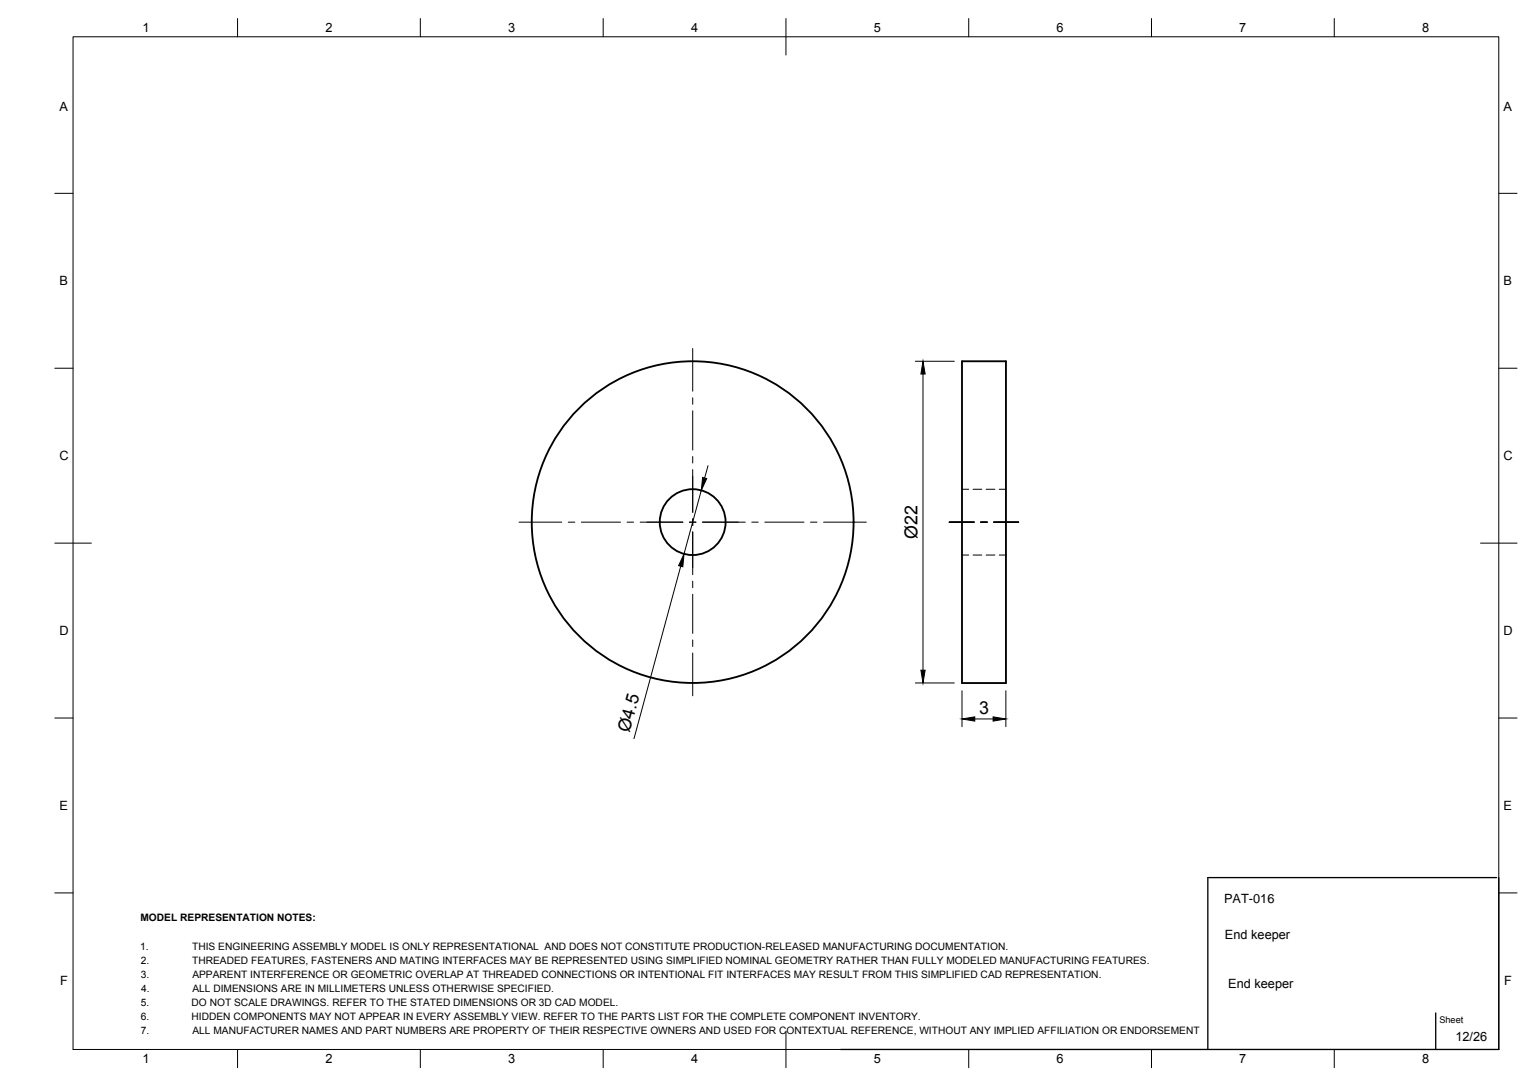
ISO-10303-21;
HEADER;
/* Generated by software containing ST-Developer
 * from STEP Tools, Inc. (www.steptools.com) 
 */

FILE_DESCRIPTION(
/* description */ ('Bracket-mounted idler roller'),
/* implementation_level */ '2;1');

FILE_NAME(
/* name */ 'End keeper.step',
/* time_stamp */ '2026-10-28T03:26:42-07:00',
/* author */ (''),
/* organization */ (''),
/* preprocessor_version */ 'ST-DEVELOPER v20.2',
/* originating_system */ 'Autodesk Translation Framework v15.17.0.0',
/* authorisation */ '');

FILE_SCHEMA (('AUTOMOTIVE_DESIGN { 1 0 10303 214 3 1 1 }'));
ENDSEC;

DATA;
#10=MECHANICAL_DESIGN_GEOMETRIC_PRESENTATION_REPRESENTATION('',(#289),#6241);
#247=SHAPE_REPRESENTATION_RELATIONSHIP('SRR','None',#6351,#268);
#268=ADVANCED_BREP_SHAPE_REPRESENTATION('',(#317),#6227);
#289=STYLED_ITEM('',(#6552),#317);
#317=MANIFOLD_SOLID_BREP('Body1',#3192);
#369=FACE_BOUND('',#826,.T.);
#370=FACE_BOUND('',#828,.T.);
#474=PLANE('',#3595);
#475=PLANE('',#3596);
#599=FACE_OUTER_BOUND('',#823,.T.);
#600=FACE_OUTER_BOUND('',#824,.T.);
#601=FACE_OUTER_BOUND('',#825,.T.);
#602=FACE_OUTER_BOUND('',#827,.T.);
#823=EDGE_LOOP('',(#2496,#2497,#2498,#2499));
#824=EDGE_LOOP('',(#2500,#2501,#2502,#2503));
#825=EDGE_LOOP('',(#2504));
#826=EDGE_LOOP('',(#2505));
#827=EDGE_LOOP('',(#2506));
#828=EDGE_LOOP('',(#2507));
#1095=LINE('',#5323,#1277);
#1096=LINE('',#5329,#1278);
#1277=VECTOR('',#4294,0.225);
#1278=VECTOR('',#4301,1.1);
#1392=CIRCLE('',#3590,0.225);
#1393=CIRCLE('',#3591,0.225);
#1394=CIRCLE('',#3593,1.1);
#1395=CIRCLE('',#3594,1.1);
#1633=VERTEX_POINT('',#5320);
#1634=VERTEX_POINT('',#5322);
#1635=VERTEX_POINT('',#5326);
#1636=VERTEX_POINT('',#5328);
#1950=EDGE_CURVE('',#1633,#1633,#1392,.T.);
#1951=EDGE_CURVE('',#1633,#1634,#1095,.T.);
#1952=EDGE_CURVE('',#1634,#1634,#1393,.T.);
#1953=EDGE_CURVE('',#1635,#1635,#1394,.T.);
#1954=EDGE_CURVE('',#1635,#1636,#1096,.T.);
#1955=EDGE_CURVE('',#1636,#1636,#1395,.T.);
#2496=ORIENTED_EDGE('',*,*,#1950,.F.);
#2497=ORIENTED_EDGE('',*,*,#1951,.T.);
#2498=ORIENTED_EDGE('',*,*,#1952,.T.);
#2499=ORIENTED_EDGE('',*,*,#1951,.F.);
#2500=ORIENTED_EDGE('',*,*,#1953,.F.);
#2501=ORIENTED_EDGE('',*,*,#1954,.T.);
#2502=ORIENTED_EDGE('',*,*,#1955,.T.);
#2503=ORIENTED_EDGE('',*,*,#1954,.F.);
#2504=ORIENTED_EDGE('',*,*,#1953,.T.);
#2505=ORIENTED_EDGE('',*,*,#1950,.T.);
#2506=ORIENTED_EDGE('',*,*,#1955,.F.);
#2507=ORIENTED_EDGE('',*,*,#1952,.F.);
#2951=CYLINDRICAL_SURFACE('',#3589,0.225);
#2952=CYLINDRICAL_SURFACE('',#3592,1.1);
#3074=ADVANCED_FACE('',(#599),#2951,.F.);
#3075=ADVANCED_FACE('',(#600),#2952,.T.);
#3076=ADVANCED_FACE('',(#601,#369),#474,.T.);
#3077=ADVANCED_FACE('',(#602,#370),#475,.F.);
#3192=CLOSED_SHELL('',(#3074,#3075,#3076,#3077));
#3588=AXIS2_PLACEMENT_3D('',#5318,#4288,#4289);
#3589=AXIS2_PLACEMENT_3D('',#5319,#4290,#4291);
#3590=AXIS2_PLACEMENT_3D('',#5321,#4292,#4293);
#3591=AXIS2_PLACEMENT_3D('',#5324,#4295,#4296);
#3592=AXIS2_PLACEMENT_3D('',#5325,#4297,#4298);
#3593=AXIS2_PLACEMENT_3D('',#5327,#4299,#4300);
#3594=AXIS2_PLACEMENT_3D('',#5330,#4302,#4303);
#3595=AXIS2_PLACEMENT_3D('',#5331,#4304,#4305);
#3596=AXIS2_PLACEMENT_3D('',#5332,#4306,#4307);
#4288=DIRECTION('axis',(0.,0.,1.));
#4289=DIRECTION('refdir',(1.,0.,0.));
#4290=DIRECTION('center_axis',(0.,1.,0.));
#4291=DIRECTION('ref_axis',(1.,0.,0.));
#4292=DIRECTION('center_axis',(0.,-1.,0.));
#4293=DIRECTION('ref_axis',(1.,0.,0.));
#4294=DIRECTION('',(0.,-1.,0.));
#4295=DIRECTION('center_axis',(0.,-1.,0.));
#4296=DIRECTION('ref_axis',(1.,0.,0.));
#4297=DIRECTION('center_axis',(0.,1.,0.));
#4298=DIRECTION('ref_axis',(1.,0.,0.));
#4299=DIRECTION('center_axis',(0.,1.,0.));
#4300=DIRECTION('ref_axis',(1.,0.,0.));
#4301=DIRECTION('',(0.,-1.,0.));
#4302=DIRECTION('center_axis',(0.,1.,0.));
#4303=DIRECTION('ref_axis',(1.,0.,0.));
#4304=DIRECTION('center_axis',(0.,1.,0.));
#4305=DIRECTION('ref_axis',(1.,0.,0.));
#4306=DIRECTION('center_axis',(0.,1.,0.));
#4307=DIRECTION('ref_axis',(1.,0.,0.));
#5318=CARTESIAN_POINT('',(0.,0.,0.));
#5319=CARTESIAN_POINT('Origin',(0.,-2.8,4.5));
#5320=CARTESIAN_POINT('',(-0.225,-2.5,4.5));
#5321=CARTESIAN_POINT('Origin',(0.,-2.5,4.5));
#5322=CARTESIAN_POINT('',(-0.225,-2.8,4.5));
#5323=CARTESIAN_POINT('',(-0.225,-2.8,4.5));
#5324=CARTESIAN_POINT('Origin',(0.,-2.8,4.5));
#5325=CARTESIAN_POINT('Origin',(0.,-2.8,4.5));
#5326=CARTESIAN_POINT('',(-1.1,-2.5,4.5));
#5327=CARTESIAN_POINT('Origin',(0.,-2.5,4.5));
#5328=CARTESIAN_POINT('',(-1.1,-2.8,4.5));
#5329=CARTESIAN_POINT('',(-1.1,-2.8,4.5));
#5330=CARTESIAN_POINT('Origin',(0.,-2.8,4.5));
#5331=CARTESIAN_POINT('Origin',(0.,-2.5,4.5));
#5332=CARTESIAN_POINT('Origin',(0.,-2.8,4.5));
#6201=UNCERTAINTY_MEASURE_WITH_UNIT(LENGTH_MEASURE(0.001),#6242,
'DISTANCE_ACCURACY_VALUE',
'Maximum model space distance between geometric entities at asserted c
onnectivities');
#6215=UNCERTAINTY_MEASURE_WITH_UNIT(LENGTH_MEASURE(0.001),#6242,
'DISTANCE_ACCURACY_VALUE',
'Maximum model space distance between geometric entities at asserted c
onnectivities');
#6227=(
GEOMETRIC_REPRESENTATION_CONTEXT(3)
GLOBAL_UNCERTAINTY_ASSIGNED_CONTEXT((#6201))
GLOBAL_UNIT_ASSIGNED_CONTEXT((#6242,#6244,#6245))
REPRESENTATION_CONTEXT('','3D')
);
#6241=(
GEOMETRIC_REPRESENTATION_CONTEXT(3)
GLOBAL_UNCERTAINTY_ASSIGNED_CONTEXT((#6215))
GLOBAL_UNIT_ASSIGNED_CONTEXT((#6242,#6244,#6245))
REPRESENTATION_CONTEXT('','3D')
);
#6242=(
LENGTH_UNIT()
NAMED_UNIT(*)
SI_UNIT(.CENTI.,.METRE.)
);
#6244=(
NAMED_UNIT(*)
PLANE_ANGLE_UNIT()
SI_UNIT($,.RADIAN.)
);
#6245=(
NAMED_UNIT(*)
SI_UNIT($,.STERADIAN.)
SOLID_ANGLE_UNIT()
);
#6257=SHAPE_DEFINITION_REPRESENTATION(#6282,#6351);
#6282=PRODUCT_DEFINITION_SHAPE('',$,#6377);
#6351=SHAPE_REPRESENTATION('',(#3588),#6227);
#6365=PRODUCT_DEFINITION_CONTEXT('part definition',#6442,'design');
#6377=PRODUCT_DEFINITION('End keeper','End keeper',#6402,#6365);
#6402=PRODUCT_DEFINITION_FORMATION('',$,#6455);
#6442=APPLICATION_CONTEXT(
'Core Data for Automotive Mechanical Design Process');
#6443=PRODUCT_CONTEXT('part definition',#6442,'mechanical');
#6455=PRODUCT('End keeper','End keeper','End keeper',(#6443));
#6546=COLOUR_RGB('Off White',0.89,0.88,0.83);
#6547=FILL_AREA_STYLE_COLOUR('',#6546);
#6548=FILL_AREA_STYLE('',(#6547));
#6549=SURFACE_STYLE_FILL_AREA(#6548);
#6550=SURFACE_SIDE_STYLE('',(#6549));
#6551=SURFACE_STYLE_USAGE(.BOTH.,#6550);
#6552=PRESENTATION_STYLE_ASSIGNMENT((#6551));
ENDSEC;
END-ISO-10303-21;
